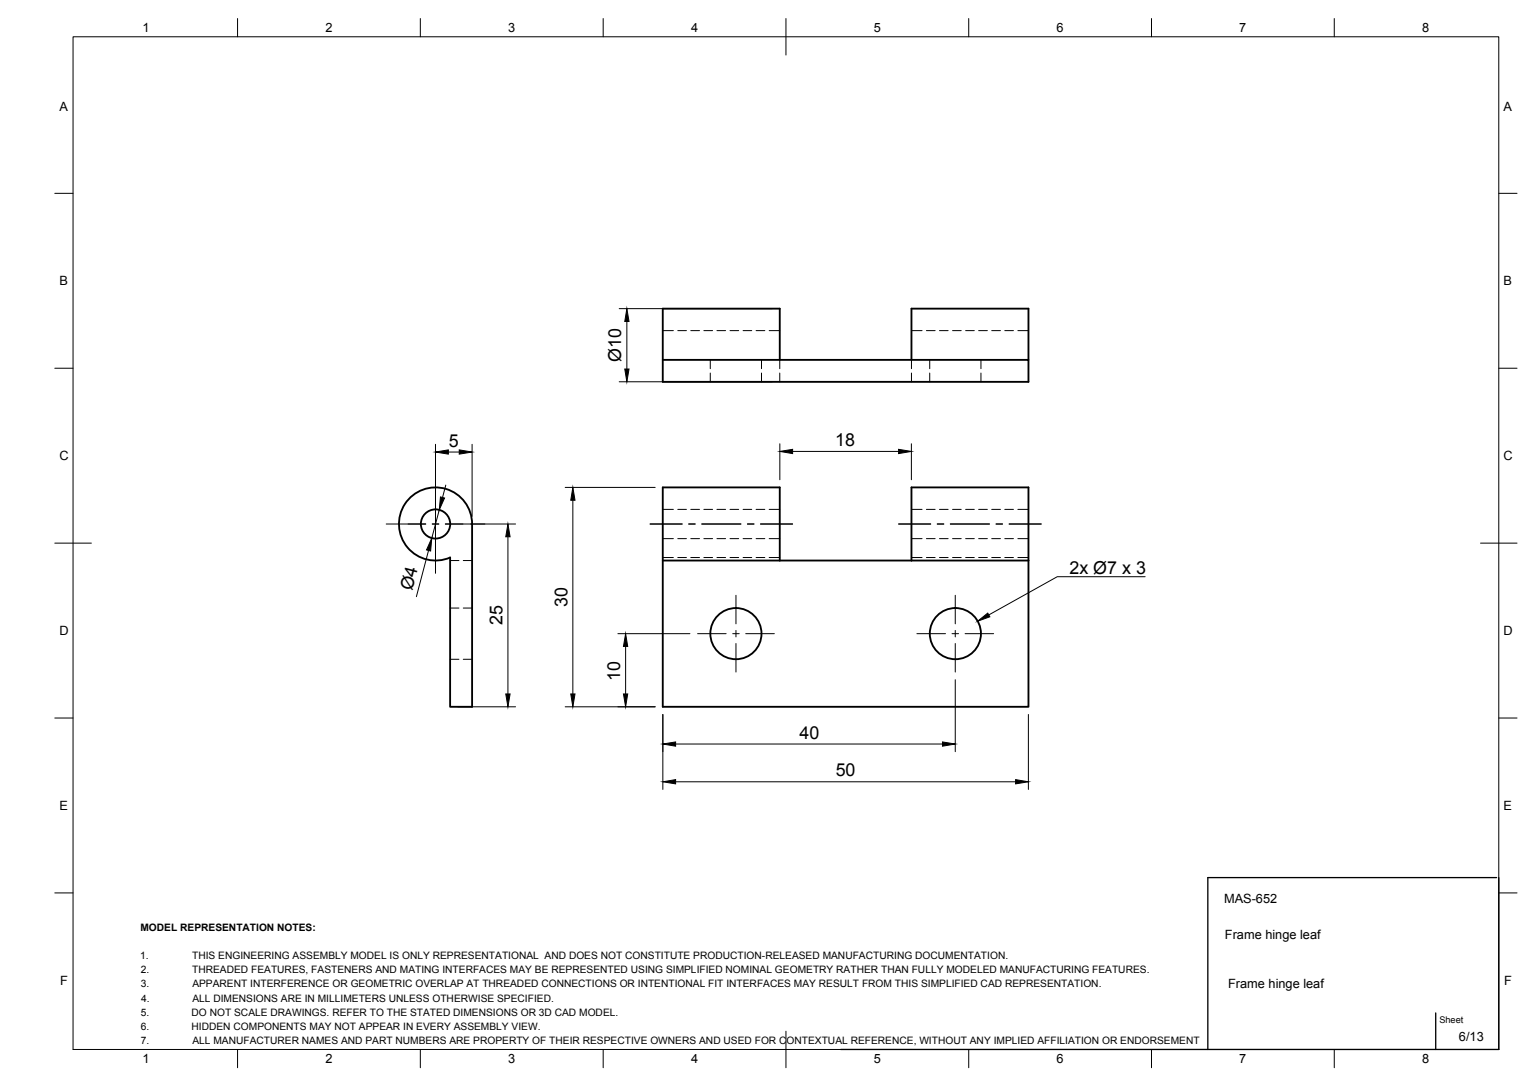
ISO-10303-21;
HEADER;
/* Generated by software containing ST-Developer
 * from STEP Tools, Inc. (www.steptools.com) 
 */

FILE_DESCRIPTION(
/* description */ ('Independent hinged machine back cover with retained hinge pins, perim
eter gasket and quarter-turn cam latch. Nominal cover 360 x 260 x 3 mm
, frame 430 x 300 x 20 mm. No guarding, structural or ingress rating a
ssigned.'),
/* implementation_level */ '2;1');

FILE_NAME(
/* name */ 'Frame hinge leaf.step',
/* time_stamp */ '2026-11-09T19:36:59-08:00',
/* author */ (''),
/* organization */ (''),
/* preprocessor_version */ 'ST-DEVELOPER v20.2',
/* originating_system */ 'Autodesk Translation Framework v15.17.0.0',
/* authorisation */ '');

FILE_SCHEMA (('AUTOMOTIVE_DESIGN { 1 0 10303 214 3 1 1 }'));
ENDSEC;

DATA;
#10=MECHANICAL_DESIGN_GEOMETRIC_PRESENTATION_REPRESENTATION('',(#207),#32627);
#171=SHAPE_REPRESENTATION_RELATIONSHIP('SRR','None',#32717,#189);
#189=ADVANCED_BREP_SHAPE_REPRESENTATION('',(#225),#32618);
#207=STYLED_ITEM('',(#32810),#225);
#225=MANIFOLD_SOLID_BREP('Body1',#8684);
#266=FACE_BOUND('',#1272,.T.);
#267=FACE_BOUND('',#1273,.T.);
#268=FACE_BOUND('',#1279,.T.);
#269=FACE_BOUND('',#1281,.T.);
#270=FACE_BOUND('',#1285,.T.);
#271=FACE_BOUND('',#1287,.T.);
#272=FACE_BOUND('',#1290,.T.);
#273=FACE_BOUND('',#1291,.T.);
#394=PLANE('',#9268);
#395=PLANE('',#9269);
#396=PLANE('',#9282);
#397=PLANE('',#9283);
#398=PLANE('',#9290);
#399=PLANE('',#9291);
#400=PLANE('',#9292);
#401=PLANE('',#9293);
#763=FACE_OUTER_BOUND('',#1270,.T.);
#764=FACE_OUTER_BOUND('',#1271,.T.);
#765=FACE_OUTER_BOUND('',#1274,.T.);
#766=FACE_OUTER_BOUND('',#1275,.T.);
#767=FACE_OUTER_BOUND('',#1276,.T.);
#768=FACE_OUTER_BOUND('',#1277,.T.);
#769=FACE_OUTER_BOUND('',#1278,.T.);
#770=FACE_OUTER_BOUND('',#1280,.T.);
#771=FACE_OUTER_BOUND('',#1282,.T.);
#772=FACE_OUTER_BOUND('',#1283,.T.);
#773=FACE_OUTER_BOUND('',#1284,.T.);
#774=FACE_OUTER_BOUND('',#1286,.T.);
#775=FACE_OUTER_BOUND('',#1288,.T.);
#776=FACE_OUTER_BOUND('',#1289,.T.);
#1270=EDGE_LOOP('',(#7053,#7054,#7055,#7056));
#1271=EDGE_LOOP('',(#7057,#7058,#7059,#7060,#7061,#7062,#7063,#7064));
#1272=EDGE_LOOP('',(#7065));
#1273=EDGE_LOOP('',(#7066));
#1274=EDGE_LOOP('',(#7067,#7068,#7069,#7070));
#1275=EDGE_LOOP('',(#7071,#7072,#7073,#7074));
#1276=EDGE_LOOP('',(#7075,#7076,#7077,#7078));
#1277=EDGE_LOOP('',(#7079,#7080,#7081,#7082));
#1278=EDGE_LOOP('',(#7083,#7084,#7085,#7086));
#1279=EDGE_LOOP('',(#7087));
#1280=EDGE_LOOP('',(#7088,#7089,#7090,#7091));
#1281=EDGE_LOOP('',(#7092));
#1282=EDGE_LOOP('',(#7093,#7094,#7095,#7096));
#1283=EDGE_LOOP('',(#7097,#7098,#7099,#7100));
#1284=EDGE_LOOP('',(#7101,#7102,#7103,#7104));
#1285=EDGE_LOOP('',(#7105));
#1286=EDGE_LOOP('',(#7106,#7107,#7108,#7109));
#1287=EDGE_LOOP('',(#7110));
#1288=EDGE_LOOP('',(#7111,#7112,#7113,#7114));
#1289=EDGE_LOOP('',(#7115,#7116,#7117,#7118,#7119,#7120,#7121,#7122));
#1290=EDGE_LOOP('',(#7123));
#1291=EDGE_LOOP('',(#7124));
#1527=CIRCLE('',#9270,3.5);
#1528=CIRCLE('',#9271,3.5);
#1529=CIRCLE('',#9273,3.5);
#1530=CIRCLE('',#9275,3.5);
#1531=CIRCLE('',#9277,5.);
#1532=CIRCLE('',#9278,5.);
#1533=CIRCLE('',#9280,2.);
#1534=CIRCLE('',#9281,2.);
#1535=CIRCLE('',#9284,5.);
#1536=CIRCLE('',#9285,2.);
#1537=CIRCLE('',#9287,2.);
#1538=CIRCLE('',#9289,5.);
#2528=LINE('',#26184,#3074);
#2529=LINE('',#26186,#3075);
#2530=LINE('',#26188,#3076);
#2531=LINE('',#26189,#3077);
#2532=LINE('',#26192,#3078);
#2533=LINE('',#26194,#3079);
#2534=LINE('',#26196,#3080);
#2535=LINE('',#26198,#3081);
#2536=LINE('',#26200,#3082);
#2537=LINE('',#26202,#3083);
#2538=LINE('',#26203,#3084);
#2539=LINE('',#26210,#3085);
#2540=LINE('',#26214,#3086);
#2541=LINE('',#26219,#3087);
#2542=LINE('',#26226,#3088);
#2543=LINE('',#26229,#3089);
#2544=LINE('',#26232,#3090);
#2545=LINE('',#26238,#3091);
#2546=LINE('',#26242,#3092);
#2547=LINE('',#26246,#3093);
#2548=LINE('',#26247,#3094);
#2549=LINE('',#26250,#3095);
#2550=LINE('',#26251,#3096);
#2551=LINE('',#26253,#3097);
#3074=VECTOR('',#10636,10.);
#3075=VECTOR('',#10637,10.);
#3076=VECTOR('',#10638,10.);
#3077=VECTOR('',#10639,10.);
#3078=VECTOR('',#10642,10.);
#3079=VECTOR('',#10643,10.);
#3080=VECTOR('',#10644,10.);
#3081=VECTOR('',#10645,10.);
#3082=VECTOR('',#10646,10.);
#3083=VECTOR('',#10647,10.);
#3084=VECTOR('',#10648,10.);
#3085=VECTOR('',#10655,3.5);
#3086=VECTOR('',#10660,3.5);
#3087=VECTOR('',#10665,10.);
#3088=VECTOR('',#10674,2.);
#3089=VECTOR('',#10679,10.);
#3090=VECTOR('',#10682,10.);
#3091=VECTOR('',#10689,2.);
#3092=VECTOR('',#10694,10.);
#3093=VECTOR('',#10699,10.);
#3094=VECTOR('',#10700,10.);
#3095=VECTOR('',#10703,10.);
#3096=VECTOR('',#10704,10.);
#3097=VECTOR('',#10707,10.);
#3829=VERTEX_POINT('',#26182);
#3830=VERTEX_POINT('',#26183);
#3831=VERTEX_POINT('',#26185);
#3832=VERTEX_POINT('',#26187);
#3833=VERTEX_POINT('',#26191);
#3834=VERTEX_POINT('',#26193);
#3835=VERTEX_POINT('',#26195);
#3836=VERTEX_POINT('',#26197);
#3837=VERTEX_POINT('',#26199);
#3838=VERTEX_POINT('',#26201);
#3839=VERTEX_POINT('',#26204);
#3840=VERTEX_POINT('',#26206);
#3841=VERTEX_POINT('',#26209);
#3842=VERTEX_POINT('',#26213);
#3843=VERTEX_POINT('',#26217);
#3844=VERTEX_POINT('',#26218);
#3845=VERTEX_POINT('',#26223);
#3846=VERTEX_POINT('',#26225);
#3847=VERTEX_POINT('',#26231);
#3848=VERTEX_POINT('',#26234);
#3849=VERTEX_POINT('',#26237);
#3850=VERTEX_POINT('',#26241);
#3851=VERTEX_POINT('',#26245);
#3852=VERTEX_POINT('',#26249);
#4950=EDGE_CURVE('',#3829,#3830,#2528,.T.);
#4951=EDGE_CURVE('',#3829,#3831,#2529,.T.);
#4952=EDGE_CURVE('',#3832,#3831,#2530,.T.);
#4953=EDGE_CURVE('',#3830,#3832,#2531,.T.);
#4954=EDGE_CURVE('',#3833,#3829,#2532,.T.);
#4955=EDGE_CURVE('',#3830,#3834,#2533,.T.);
#4956=EDGE_CURVE('',#3834,#3835,#2534,.T.);
#4957=EDGE_CURVE('',#3835,#3836,#2535,.T.);
#4958=EDGE_CURVE('',#3836,#3837,#2536,.T.);
#4959=EDGE_CURVE('',#3837,#3838,#2537,.T.);
#4960=EDGE_CURVE('',#3838,#3833,#2538,.T.);
#4961=EDGE_CURVE('',#3839,#3839,#1527,.T.);
#4962=EDGE_CURVE('',#3840,#3840,#1528,.T.);
#4963=EDGE_CURVE('',#3840,#3841,#2539,.T.);
#4964=EDGE_CURVE('',#3841,#3841,#1529,.T.);
#4965=EDGE_CURVE('',#3839,#3842,#2540,.T.);
#4966=EDGE_CURVE('',#3842,#3842,#1530,.T.);
#4967=EDGE_CURVE('',#3843,#3844,#2541,.T.);
#4968=EDGE_CURVE('',#3835,#3843,#1531,.T.);
#4969=EDGE_CURVE('',#3834,#3844,#1532,.T.);
#4970=EDGE_CURVE('',#3845,#3845,#1533,.T.);
#4971=EDGE_CURVE('',#3845,#3846,#2542,.T.);
#4972=EDGE_CURVE('',#3846,#3846,#1534,.T.);
#4973=EDGE_CURVE('',#3844,#3832,#2543,.T.);
#4974=EDGE_CURVE('',#3831,#3847,#2544,.T.);
#4975=EDGE_CURVE('',#3833,#3847,#1535,.T.);
#4976=EDGE_CURVE('',#3848,#3848,#1536,.T.);
#4977=EDGE_CURVE('',#3848,#3849,#2545,.T.);
#4978=EDGE_CURVE('',#3849,#3849,#1537,.T.);
#4979=EDGE_CURVE('',#3847,#3850,#2546,.T.);
#4980=EDGE_CURVE('',#3838,#3850,#1538,.T.);
#4981=EDGE_CURVE('',#3851,#3837,#2547,.T.);
#4982=EDGE_CURVE('',#3851,#3850,#2548,.T.);
#4983=EDGE_CURVE('',#3843,#3852,#2549,.T.);
#4984=EDGE_CURVE('',#3852,#3836,#2550,.T.);
#4985=EDGE_CURVE('',#3852,#3851,#2551,.T.);
#7053=ORIENTED_EDGE('',*,*,#4950,.F.);
#7054=ORIENTED_EDGE('',*,*,#4951,.T.);
#7055=ORIENTED_EDGE('',*,*,#4952,.F.);
#7056=ORIENTED_EDGE('',*,*,#4953,.F.);
#7057=ORIENTED_EDGE('',*,*,#4954,.T.);
#7058=ORIENTED_EDGE('',*,*,#4950,.T.);
#7059=ORIENTED_EDGE('',*,*,#4955,.T.);
#7060=ORIENTED_EDGE('',*,*,#4956,.T.);
#7061=ORIENTED_EDGE('',*,*,#4957,.T.);
#7062=ORIENTED_EDGE('',*,*,#4958,.T.);
#7063=ORIENTED_EDGE('',*,*,#4959,.T.);
#7064=ORIENTED_EDGE('',*,*,#4960,.T.);
#7065=ORIENTED_EDGE('',*,*,#4961,.T.);
#7066=ORIENTED_EDGE('',*,*,#4962,.T.);
#7067=ORIENTED_EDGE('',*,*,#4962,.F.);
#7068=ORIENTED_EDGE('',*,*,#4963,.T.);
#7069=ORIENTED_EDGE('',*,*,#4964,.F.);
#7070=ORIENTED_EDGE('',*,*,#4963,.F.);
#7071=ORIENTED_EDGE('',*,*,#4961,.F.);
#7072=ORIENTED_EDGE('',*,*,#4965,.T.);
#7073=ORIENTED_EDGE('',*,*,#4966,.F.);
#7074=ORIENTED_EDGE('',*,*,#4965,.F.);
#7075=ORIENTED_EDGE('',*,*,#4967,.F.);
#7076=ORIENTED_EDGE('',*,*,#4968,.F.);
#7077=ORIENTED_EDGE('',*,*,#4956,.F.);
#7078=ORIENTED_EDGE('',*,*,#4969,.T.);
#7079=ORIENTED_EDGE('',*,*,#4970,.F.);
#7080=ORIENTED_EDGE('',*,*,#4971,.T.);
#7081=ORIENTED_EDGE('',*,*,#4972,.T.);
#7082=ORIENTED_EDGE('',*,*,#4971,.F.);
#7083=ORIENTED_EDGE('',*,*,#4969,.F.);
#7084=ORIENTED_EDGE('',*,*,#4955,.F.);
#7085=ORIENTED_EDGE('',*,*,#4953,.T.);
#7086=ORIENTED_EDGE('',*,*,#4973,.F.);
#7087=ORIENTED_EDGE('',*,*,#4972,.F.);
#7088=ORIENTED_EDGE('',*,*,#4974,.F.);
#7089=ORIENTED_EDGE('',*,*,#4951,.F.);
#7090=ORIENTED_EDGE('',*,*,#4954,.F.);
#7091=ORIENTED_EDGE('',*,*,#4975,.T.);
#7092=ORIENTED_EDGE('',*,*,#4976,.T.);
#7093=ORIENTED_EDGE('',*,*,#4976,.F.);
#7094=ORIENTED_EDGE('',*,*,#4977,.T.);
#7095=ORIENTED_EDGE('',*,*,#4978,.T.);
#7096=ORIENTED_EDGE('',*,*,#4977,.F.);
#7097=ORIENTED_EDGE('',*,*,#4979,.F.);
#7098=ORIENTED_EDGE('',*,*,#4975,.F.);
#7099=ORIENTED_EDGE('',*,*,#4960,.F.);
#7100=ORIENTED_EDGE('',*,*,#4980,.T.);
#7101=ORIENTED_EDGE('',*,*,#4980,.F.);
#7102=ORIENTED_EDGE('',*,*,#4959,.F.);
#7103=ORIENTED_EDGE('',*,*,#4981,.F.);
#7104=ORIENTED_EDGE('',*,*,#4982,.T.);
#7105=ORIENTED_EDGE('',*,*,#4978,.F.);
#7106=ORIENTED_EDGE('',*,*,#4983,.T.);
#7107=ORIENTED_EDGE('',*,*,#4984,.T.);
#7108=ORIENTED_EDGE('',*,*,#4957,.F.);
#7109=ORIENTED_EDGE('',*,*,#4968,.T.);
#7110=ORIENTED_EDGE('',*,*,#4970,.T.);
#7111=ORIENTED_EDGE('',*,*,#4985,.T.);
#7112=ORIENTED_EDGE('',*,*,#4981,.T.);
#7113=ORIENTED_EDGE('',*,*,#4958,.F.);
#7114=ORIENTED_EDGE('',*,*,#4984,.F.);
#7115=ORIENTED_EDGE('',*,*,#4974,.T.);
#7116=ORIENTED_EDGE('',*,*,#4979,.T.);
#7117=ORIENTED_EDGE('',*,*,#4982,.F.);
#7118=ORIENTED_EDGE('',*,*,#4985,.F.);
#7119=ORIENTED_EDGE('',*,*,#4983,.F.);
#7120=ORIENTED_EDGE('',*,*,#4967,.T.);
#7121=ORIENTED_EDGE('',*,*,#4973,.T.);
#7122=ORIENTED_EDGE('',*,*,#4952,.T.);
#7123=ORIENTED_EDGE('',*,*,#4964,.T.);
#7124=ORIENTED_EDGE('',*,*,#4966,.T.);
#8102=CYLINDRICAL_SURFACE('',#9272,3.5);
#8103=CYLINDRICAL_SURFACE('',#9274,3.5);
#8104=CYLINDRICAL_SURFACE('',#9276,5.);
#8105=CYLINDRICAL_SURFACE('',#9279,2.);
#8106=CYLINDRICAL_SURFACE('',#9286,2.);
#8107=CYLINDRICAL_SURFACE('',#9288,5.);
#8511=ADVANCED_FACE('',(#763),#394,.F.);
#8512=ADVANCED_FACE('',(#764,#266,#267),#395,.T.);
#8513=ADVANCED_FACE('',(#765),#8102,.F.);
#8514=ADVANCED_FACE('',(#766),#8103,.F.);
#8515=ADVANCED_FACE('',(#767),#8104,.T.);
#8516=ADVANCED_FACE('',(#768),#8105,.F.);
#8517=ADVANCED_FACE('',(#769,#268),#396,.F.);
#8518=ADVANCED_FACE('',(#770,#269),#397,.T.);
#8519=ADVANCED_FACE('',(#771),#8106,.F.);
#8520=ADVANCED_FACE('',(#772),#8107,.T.);
#8521=ADVANCED_FACE('',(#773,#270),#398,.T.);
#8522=ADVANCED_FACE('',(#774,#271),#399,.T.);
#8523=ADVANCED_FACE('',(#775),#400,.T.);
#8524=ADVANCED_FACE('',(#776,#272,#273),#401,.F.);
#8684=CLOSED_SHELL('',(#8511,#8512,#8513,#8514,#8515,#8516,#8517,#8518,
#8519,#8520,#8521,#8522,#8523,#8524));
#9267=AXIS2_PLACEMENT_3D('',#26180,#10632,#10633);
#9268=AXIS2_PLACEMENT_3D('',#26181,#10634,#10635);
#9269=AXIS2_PLACEMENT_3D('',#26190,#10640,#10641);
#9270=AXIS2_PLACEMENT_3D('',#26205,#10649,#10650);
#9271=AXIS2_PLACEMENT_3D('',#26207,#10651,#10652);
#9272=AXIS2_PLACEMENT_3D('',#26208,#10653,#10654);
#9273=AXIS2_PLACEMENT_3D('',#26211,#10656,#10657);
#9274=AXIS2_PLACEMENT_3D('',#26212,#10658,#10659);
#9275=AXIS2_PLACEMENT_3D('',#26215,#10661,#10662);
#9276=AXIS2_PLACEMENT_3D('',#26216,#10663,#10664);
#9277=AXIS2_PLACEMENT_3D('',#26220,#10666,#10667);
#9278=AXIS2_PLACEMENT_3D('',#26221,#10668,#10669);
#9279=AXIS2_PLACEMENT_3D('',#26222,#10670,#10671);
#9280=AXIS2_PLACEMENT_3D('',#26224,#10672,#10673);
#9281=AXIS2_PLACEMENT_3D('',#26227,#10675,#10676);
#9282=AXIS2_PLACEMENT_3D('',#26228,#10677,#10678);
#9283=AXIS2_PLACEMENT_3D('',#26230,#10680,#10681);
#9284=AXIS2_PLACEMENT_3D('',#26233,#10683,#10684);
#9285=AXIS2_PLACEMENT_3D('',#26235,#10685,#10686);
#9286=AXIS2_PLACEMENT_3D('',#26236,#10687,#10688);
#9287=AXIS2_PLACEMENT_3D('',#26239,#10690,#10691);
#9288=AXIS2_PLACEMENT_3D('',#26240,#10692,#10693);
#9289=AXIS2_PLACEMENT_3D('',#26243,#10695,#10696);
#9290=AXIS2_PLACEMENT_3D('',#26244,#10697,#10698);
#9291=AXIS2_PLACEMENT_3D('',#26248,#10701,#10702);
#9292=AXIS2_PLACEMENT_3D('',#26252,#10705,#10706);
#9293=AXIS2_PLACEMENT_3D('',#26254,#10708,#10709);
#10632=DIRECTION('axis',(0.,0.,1.));
#10633=DIRECTION('refdir',(1.,0.,0.));
#10634=DIRECTION('center_axis',(-1.,0.,0.));
#10635=DIRECTION('ref_axis',(0.,1.,0.));
#10636=DIRECTION('',(0.,1.,0.));
#10637=DIRECTION('',(0.,0.,-1.));
#10638=DIRECTION('',(0.,-1.,0.));
#10639=DIRECTION('',(0.,0.,-1.));
#10640=DIRECTION('center_axis',(0.,0.,1.));
#10641=DIRECTION('ref_axis',(1.,0.,0.));
#10642=DIRECTION('',(-1.,0.,0.));
#10643=DIRECTION('',(1.,0.,0.));
#10644=DIRECTION('',(0.,1.,0.));
#10645=DIRECTION('',(-1.,0.,0.));
#10646=DIRECTION('',(0.,-1.,0.));
#10647=DIRECTION('',(1.,0.,0.));
#10648=DIRECTION('',(0.,1.,0.));
#10649=DIRECTION('center_axis',(0.,0.,-1.));
#10650=DIRECTION('ref_axis',(1.,0.,0.));
#10651=DIRECTION('center_axis',(0.,0.,-1.));
#10652=DIRECTION('ref_axis',(1.,0.,0.));
#10653=DIRECTION('center_axis',(0.,0.,-1.));
#10654=DIRECTION('ref_axis',(1.,0.,0.));
#10655=DIRECTION('',(0.,0.,-1.));
#10656=DIRECTION('center_axis',(0.,0.,1.));
#10657=DIRECTION('ref_axis',(1.,0.,0.));
#10658=DIRECTION('center_axis',(0.,0.,-1.));
#10659=DIRECTION('ref_axis',(1.,0.,0.));
#10660=DIRECTION('',(0.,0.,-1.));
#10661=DIRECTION('center_axis',(0.,0.,1.));
#10662=DIRECTION('ref_axis',(1.,0.,0.));
#10663=DIRECTION('center_axis',(0.,1.,0.));
#10664=DIRECTION('ref_axis',(0.547722557505166,0.,-0.836660026534075));
#10665=DIRECTION('',(0.,-1.,0.));
#10666=DIRECTION('center_axis',(0.,1.,0.));
#10667=DIRECTION('ref_axis',(1.,0.,0.));
#10668=DIRECTION('center_axis',(0.,1.,0.));
#10669=DIRECTION('ref_axis',(1.,0.,0.));
#10670=DIRECTION('center_axis',(0.,1.,0.));
#10671=DIRECTION('ref_axis',(1.,0.,0.));
#10672=DIRECTION('center_axis',(0.,-1.,0.));
#10673=DIRECTION('ref_axis',(1.,0.,0.));
#10674=DIRECTION('',(0.,-1.,0.));
#10675=DIRECTION('center_axis',(0.,-1.,0.));
#10676=DIRECTION('ref_axis',(1.,0.,0.));
#10677=DIRECTION('center_axis',(0.,1.,0.));
#10678=DIRECTION('ref_axis',(1.,0.,0.));
#10679=DIRECTION('',(-1.,0.,0.));
#10680=DIRECTION('center_axis',(0.,1.,0.));
#10681=DIRECTION('ref_axis',(1.,0.,0.));
#10682=DIRECTION('',(1.,0.,0.));
#10683=DIRECTION('center_axis',(0.,1.,0.));
#10684=DIRECTION('ref_axis',(1.,0.,0.));
#10685=DIRECTION('center_axis',(0.,-1.,0.));
#10686=DIRECTION('ref_axis',(1.,0.,0.));
#10687=DIRECTION('center_axis',(0.,1.,0.));
#10688=DIRECTION('ref_axis',(1.,0.,0.));
#10689=DIRECTION('',(0.,-1.,0.));
#10690=DIRECTION('center_axis',(0.,-1.,0.));
#10691=DIRECTION('ref_axis',(1.,0.,0.));
#10692=DIRECTION('center_axis',(0.,1.,0.));
#10693=DIRECTION('ref_axis',(0.547722557505166,0.,-0.836660026534075));
#10694=DIRECTION('',(0.,-1.,0.));
#10695=DIRECTION('center_axis',(0.,1.,0.));
#10696=DIRECTION('ref_axis',(1.,0.,0.));
#10697=DIRECTION('center_axis',(0.,-1.,0.));
#10698=DIRECTION('ref_axis',(1.,0.,0.));
#10699=DIRECTION('',(0.,0.,1.));
#10700=DIRECTION('',(1.,0.,0.));
#10701=DIRECTION('center_axis',(0.,1.,0.));
#10702=DIRECTION('ref_axis',(-1.,0.,0.));
#10703=DIRECTION('',(-1.,0.,0.));
#10704=DIRECTION('',(0.,0.,1.));
#10705=DIRECTION('center_axis',(-1.,0.,0.));
#10706=DIRECTION('ref_axis',(0.,-1.,0.));
#10707=DIRECTION('',(0.,-1.,0.));
#10708=DIRECTION('center_axis',(0.,0.,1.));
#10709=DIRECTION('ref_axis',(1.,0.,0.));
#26180=CARTESIAN_POINT('',(0.,0.,0.));
#26181=CARTESIAN_POINT('Origin',(-5.,-9.,0.));
#26182=CARTESIAN_POINT('',(-5.,-9.,0.));
#26183=CARTESIAN_POINT('',(-5.,9.,0.));
#26184=CARTESIAN_POINT('',(-5.,-4.5,0.));
#26185=CARTESIAN_POINT('',(-5.,-9.,-3.));
#26186=CARTESIAN_POINT('',(-5.,-9.,0.));
#26187=CARTESIAN_POINT('',(-5.,9.,-3.));
#26188=CARTESIAN_POINT('',(-5.,-4.5,-3.));
#26189=CARTESIAN_POINT('',(-5.,9.,0.));
#26190=CARTESIAN_POINT('Origin',(-12.5,0.,0.));
#26191=CARTESIAN_POINT('',(0.,-9.,0.));
#26192=CARTESIAN_POINT('',(-6.25,-9.,0.));
#26193=CARTESIAN_POINT('',(0.,9.,0.));
#26194=CARTESIAN_POINT('',(-8.75,9.,0.));
#26195=CARTESIAN_POINT('',(0.,25.,0.));
#26196=CARTESIAN_POINT('',(0.,-25.,0.));
#26197=CARTESIAN_POINT('',(-25.,25.,0.));
#26198=CARTESIAN_POINT('',(0.,25.,0.));
#26199=CARTESIAN_POINT('',(-25.,-25.,0.));
#26200=CARTESIAN_POINT('',(-25.,25.,0.));
#26201=CARTESIAN_POINT('',(0.,-25.,0.));
#26202=CARTESIAN_POINT('',(-25.,-25.,0.));
#26203=CARTESIAN_POINT('',(0.,-25.,0.));
#26204=CARTESIAN_POINT('',(-18.5,15.,0.));
#26205=CARTESIAN_POINT('Origin',(-15.,15.,0.));
#26206=CARTESIAN_POINT('',(-18.5,-15.,0.));
#26207=CARTESIAN_POINT('Origin',(-15.,-15.,0.));
#26208=CARTESIAN_POINT('Origin',(-15.,-15.,-1.5));
#26209=CARTESIAN_POINT('',(-18.5,-15.,-3.));
#26210=CARTESIAN_POINT('',(-18.5,-15.,-1.5));
#26211=CARTESIAN_POINT('Origin',(-15.,-15.,-3.));
#26212=CARTESIAN_POINT('Origin',(-15.,15.,-1.5));
#26213=CARTESIAN_POINT('',(-18.5,15.,-3.));
#26214=CARTESIAN_POINT('',(-18.5,15.,-1.5));
#26215=CARTESIAN_POINT('Origin',(-15.,15.,-3.));
#26216=CARTESIAN_POINT('Origin',(0.,9.,-5.));
#26217=CARTESIAN_POINT('',(-4.58257569495584,25.,-3.));
#26218=CARTESIAN_POINT('',(-4.58257569495584,9.,-3.));
#26219=CARTESIAN_POINT('',(-4.58257569495584,9.,-3.));
#26220=CARTESIAN_POINT('Origin',(0.,25.,-5.));
#26221=CARTESIAN_POINT('Origin',(0.,9.,-5.));
#26222=CARTESIAN_POINT('Origin',(0.,9.,-5.));
#26223=CARTESIAN_POINT('',(-2.,25.,-5.));
#26224=CARTESIAN_POINT('Origin',(0.,25.,-5.));
#26225=CARTESIAN_POINT('',(-2.,9.,-5.));
#26226=CARTESIAN_POINT('',(-2.,9.,-5.));
#26227=CARTESIAN_POINT('Origin',(0.,9.,-5.));
#26228=CARTESIAN_POINT('Origin',(0.,9.,-5.));
#26229=CARTESIAN_POINT('',(-8.75,9.,-3.));
#26230=CARTESIAN_POINT('Origin',(0.,-9.,-5.));
#26231=CARTESIAN_POINT('',(-4.58257569495584,-9.,-3.));
#26232=CARTESIAN_POINT('',(-6.25,-9.,-3.));
#26233=CARTESIAN_POINT('Origin',(0.,-9.,-5.));
#26234=CARTESIAN_POINT('',(-2.,-9.,-5.));
#26235=CARTESIAN_POINT('Origin',(0.,-9.,-5.));
#26236=CARTESIAN_POINT('Origin',(0.,-25.,-5.));
#26237=CARTESIAN_POINT('',(-2.,-25.,-5.));
#26238=CARTESIAN_POINT('',(-2.,-25.,-5.));
#26239=CARTESIAN_POINT('Origin',(0.,-25.,-5.));
#26240=CARTESIAN_POINT('Origin',(0.,-25.,-5.));
#26241=CARTESIAN_POINT('',(-4.58257569495584,-25.,-3.));
#26242=CARTESIAN_POINT('',(-4.58257569495584,-25.,-3.));
#26243=CARTESIAN_POINT('Origin',(0.,-25.,-5.));
#26244=CARTESIAN_POINT('Origin',(-25.,-25.,-3.));
#26245=CARTESIAN_POINT('',(-25.,-25.,-3.));
#26246=CARTESIAN_POINT('',(-25.,-25.,-3.));
#26247=CARTESIAN_POINT('',(-25.,-25.,-3.));
#26248=CARTESIAN_POINT('Origin',(0.,25.,-3.));
#26249=CARTESIAN_POINT('',(-25.,25.,-3.));
#26250=CARTESIAN_POINT('',(0.,25.,-3.));
#26251=CARTESIAN_POINT('',(-25.,25.,-3.));
#26252=CARTESIAN_POINT('Origin',(-25.,25.,-3.));
#26253=CARTESIAN_POINT('',(-25.,25.,-3.));
#26254=CARTESIAN_POINT('Origin',(-12.5,0.,-3.));
#32598=UNCERTAINTY_MEASURE_WITH_UNIT(LENGTH_MEASURE(0.01),#32628,
'DISTANCE_ACCURACY_VALUE',
'Maximum model space distance between geometric entities at asserted c
onnectivities');
#32607=UNCERTAINTY_MEASURE_WITH_UNIT(LENGTH_MEASURE(0.01),#32628,
'DISTANCE_ACCURACY_VALUE',
'Maximum model space distance between geometric entities at asserted c
onnectivities');
#32618=(
GEOMETRIC_REPRESENTATION_CONTEXT(3)
GLOBAL_UNCERTAINTY_ASSIGNED_CONTEXT((#32598))
GLOBAL_UNIT_ASSIGNED_CONTEXT((#32628,#32630,#32631))
REPRESENTATION_CONTEXT('','3D')
);
#32627=(
GEOMETRIC_REPRESENTATION_CONTEXT(3)
GLOBAL_UNCERTAINTY_ASSIGNED_CONTEXT((#32607))
GLOBAL_UNIT_ASSIGNED_CONTEXT((#32628,#32630,#32631))
REPRESENTATION_CONTEXT('','3D')
);
#32628=(
LENGTH_UNIT()
NAMED_UNIT(*)
SI_UNIT(.MILLI.,.METRE.)
);
#32630=(
NAMED_UNIT(*)
PLANE_ANGLE_UNIT()
SI_UNIT($,.RADIAN.)
);
#32631=(
NAMED_UNIT(*)
SI_UNIT($,.STERADIAN.)
SOLID_ANGLE_UNIT()
);
#32642=SHAPE_DEFINITION_REPRESENTATION(#32661,#32717);
#32661=PRODUCT_DEFINITION_SHAPE('',$,#32737);
#32717=SHAPE_REPRESENTATION('',(#9267),#32618);
#32726=PRODUCT_DEFINITION_CONTEXT('part definition',#32785,'design');
#32737=PRODUCT_DEFINITION('Frame hinge leaf','Frame hinge leaf',#32756,
#32726);
#32756=PRODUCT_DEFINITION_FORMATION('',$,#32797);
#32785=APPLICATION_CONTEXT(
'Core Data for Automotive Mechanical Design Process');
#32786=PRODUCT_CONTEXT('part definition',#32785,'mechanical');
#32797=PRODUCT('Frame hinge leaf','Frame hinge leaf',$,(#32786));
#32810=PRESENTATION_STYLE_ASSIGNMENT((#32817));
#32817=SURFACE_STYLE_USAGE(.BOTH.,#32824);
#32824=SURFACE_SIDE_STYLE('',(#32831));
#32831=SURFACE_STYLE_FILL_AREA(#32838);
#32838=FILL_AREA_STYLE('Gray',(#32845));
#32845=FILL_AREA_STYLE_COLOUR('Gray',#32852);
#32852=COLOUR_RGB('Gray',0.407843137254902,0.447058823529412,0.498039215686275);
ENDSEC;
END-ISO-10303-21;
